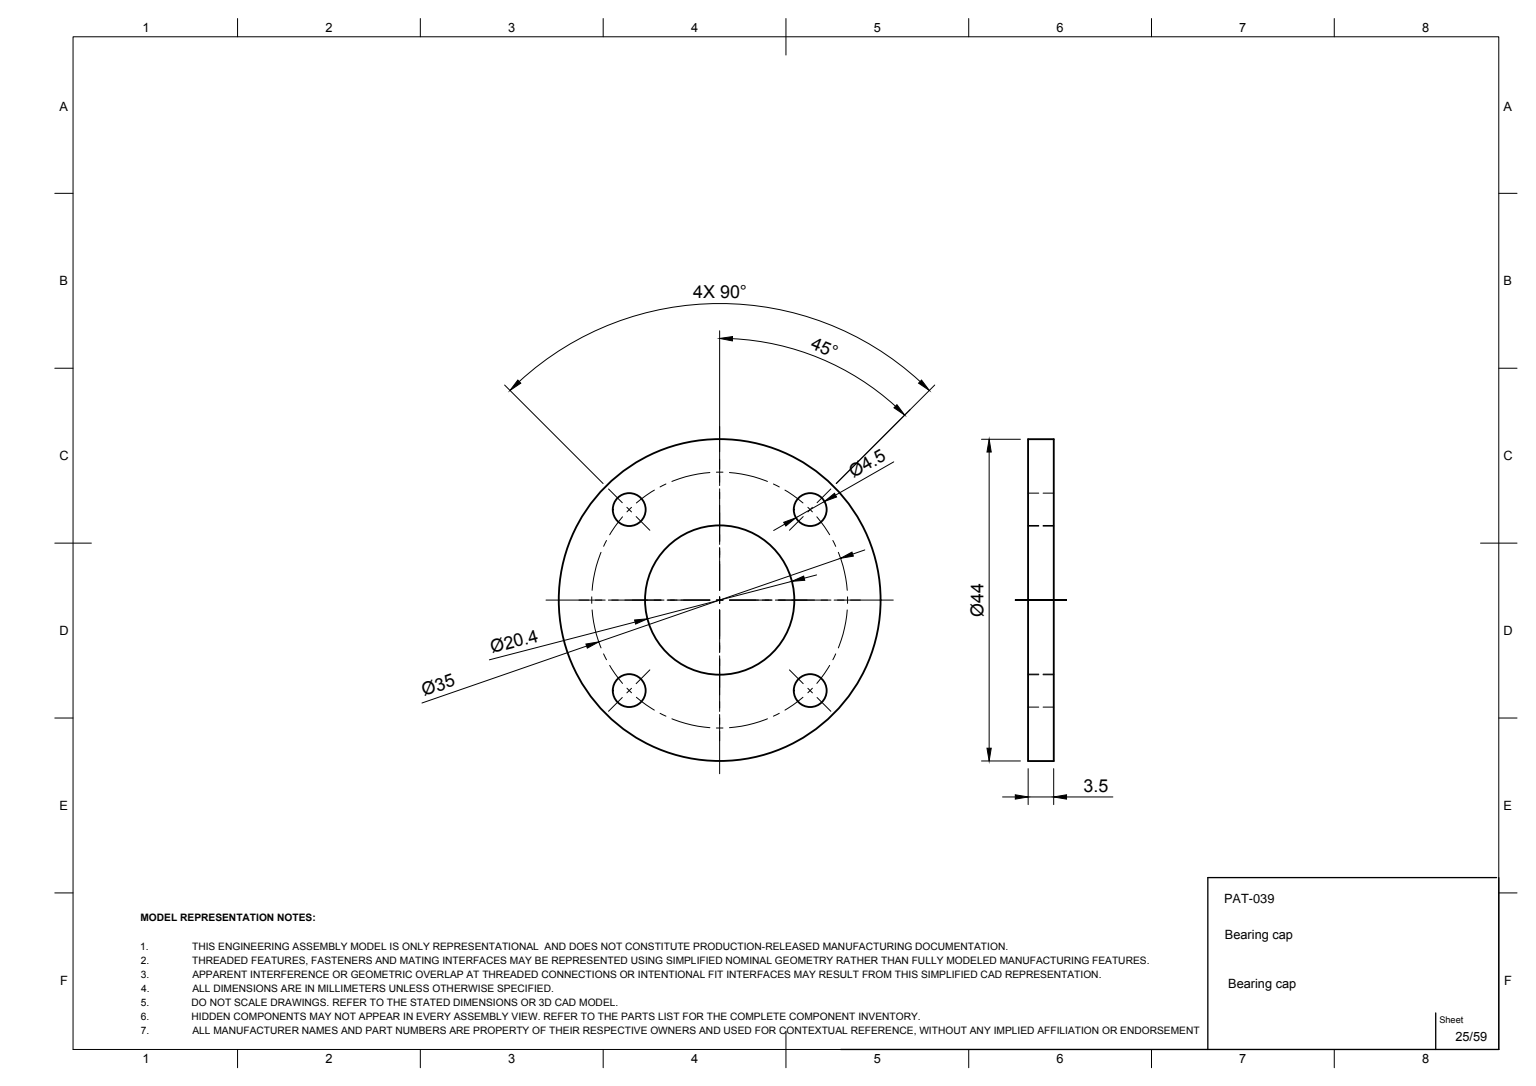
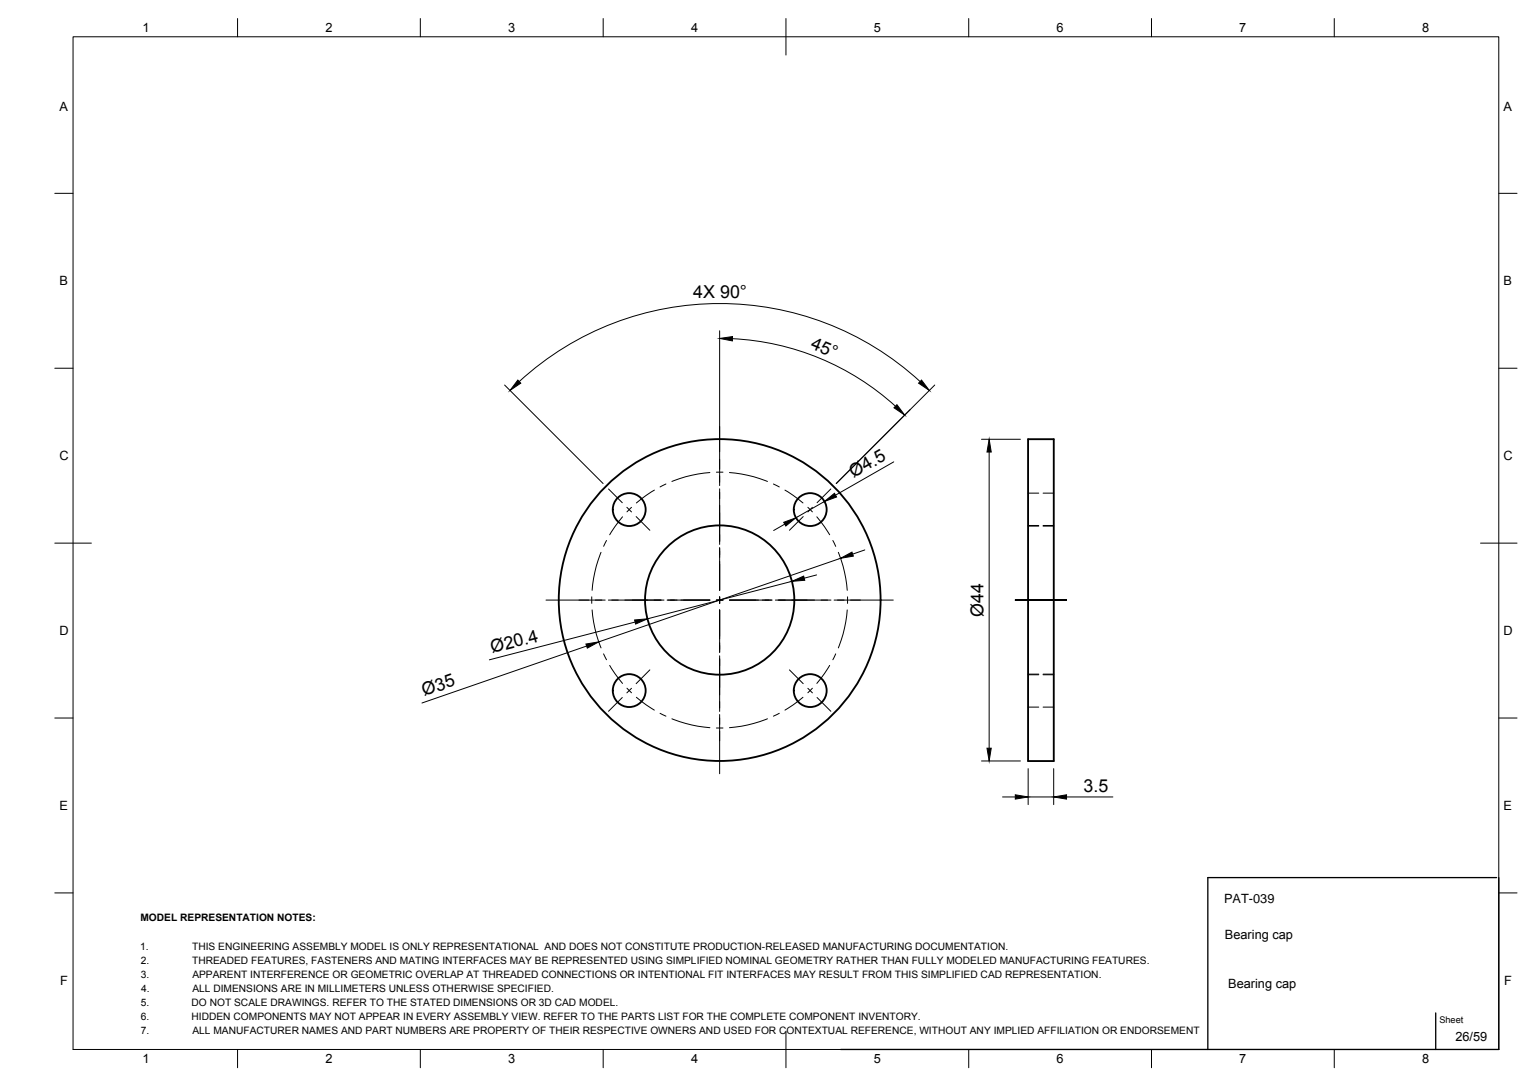
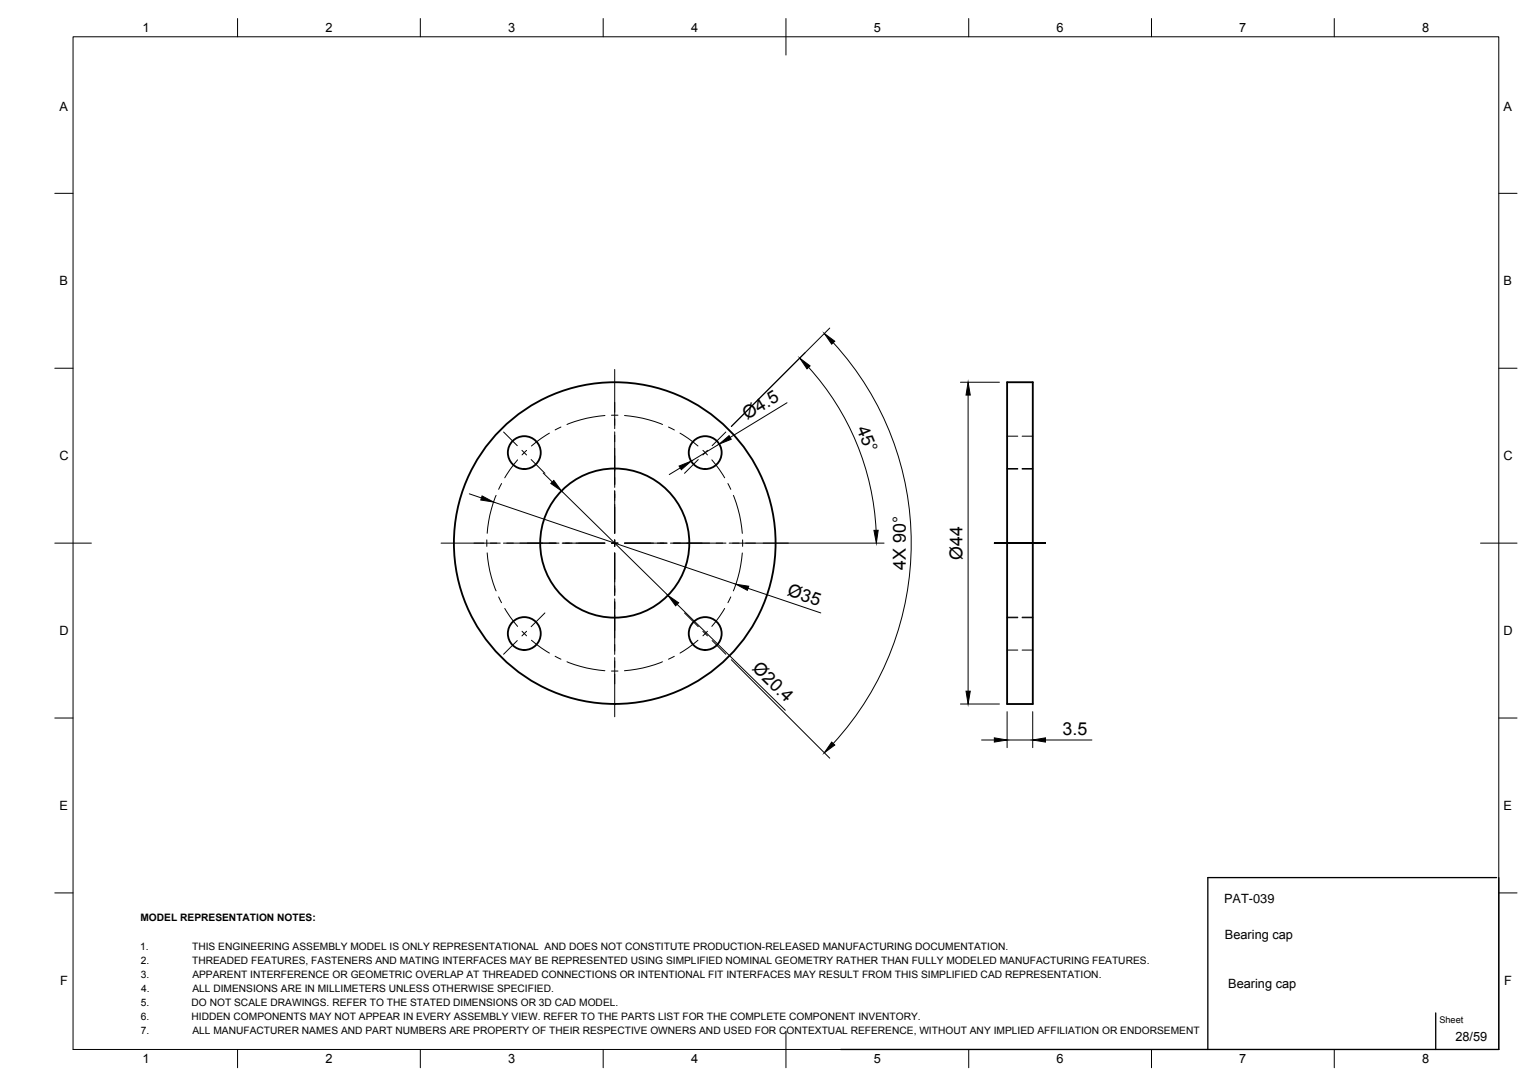
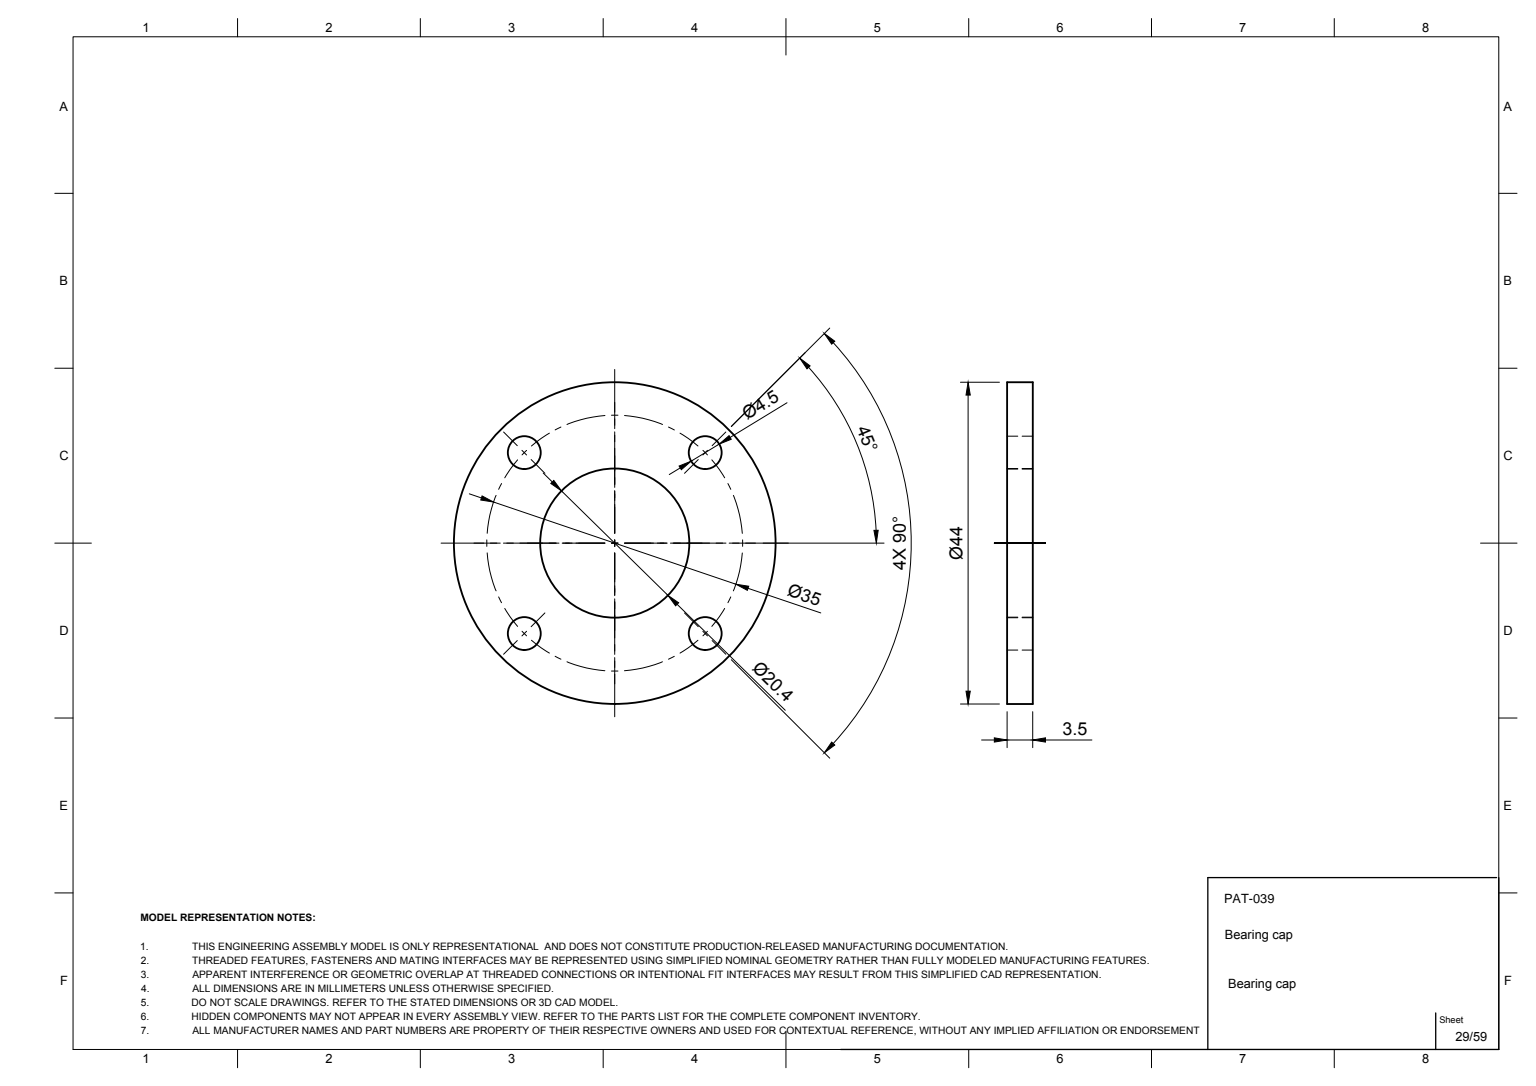
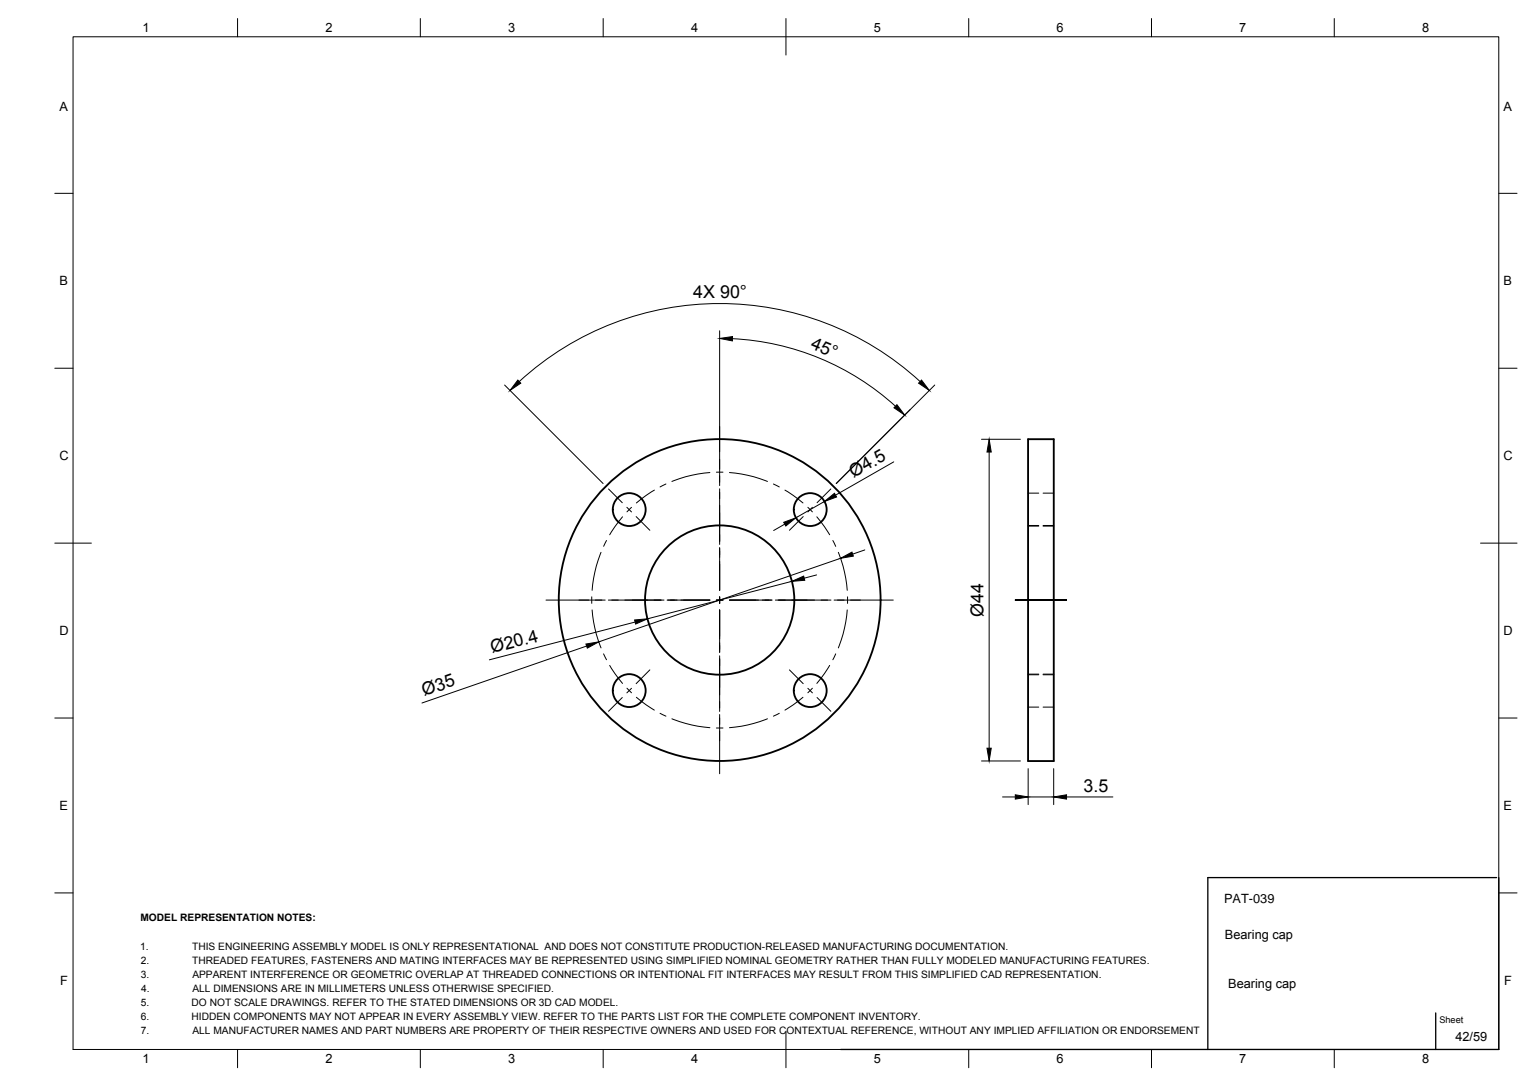
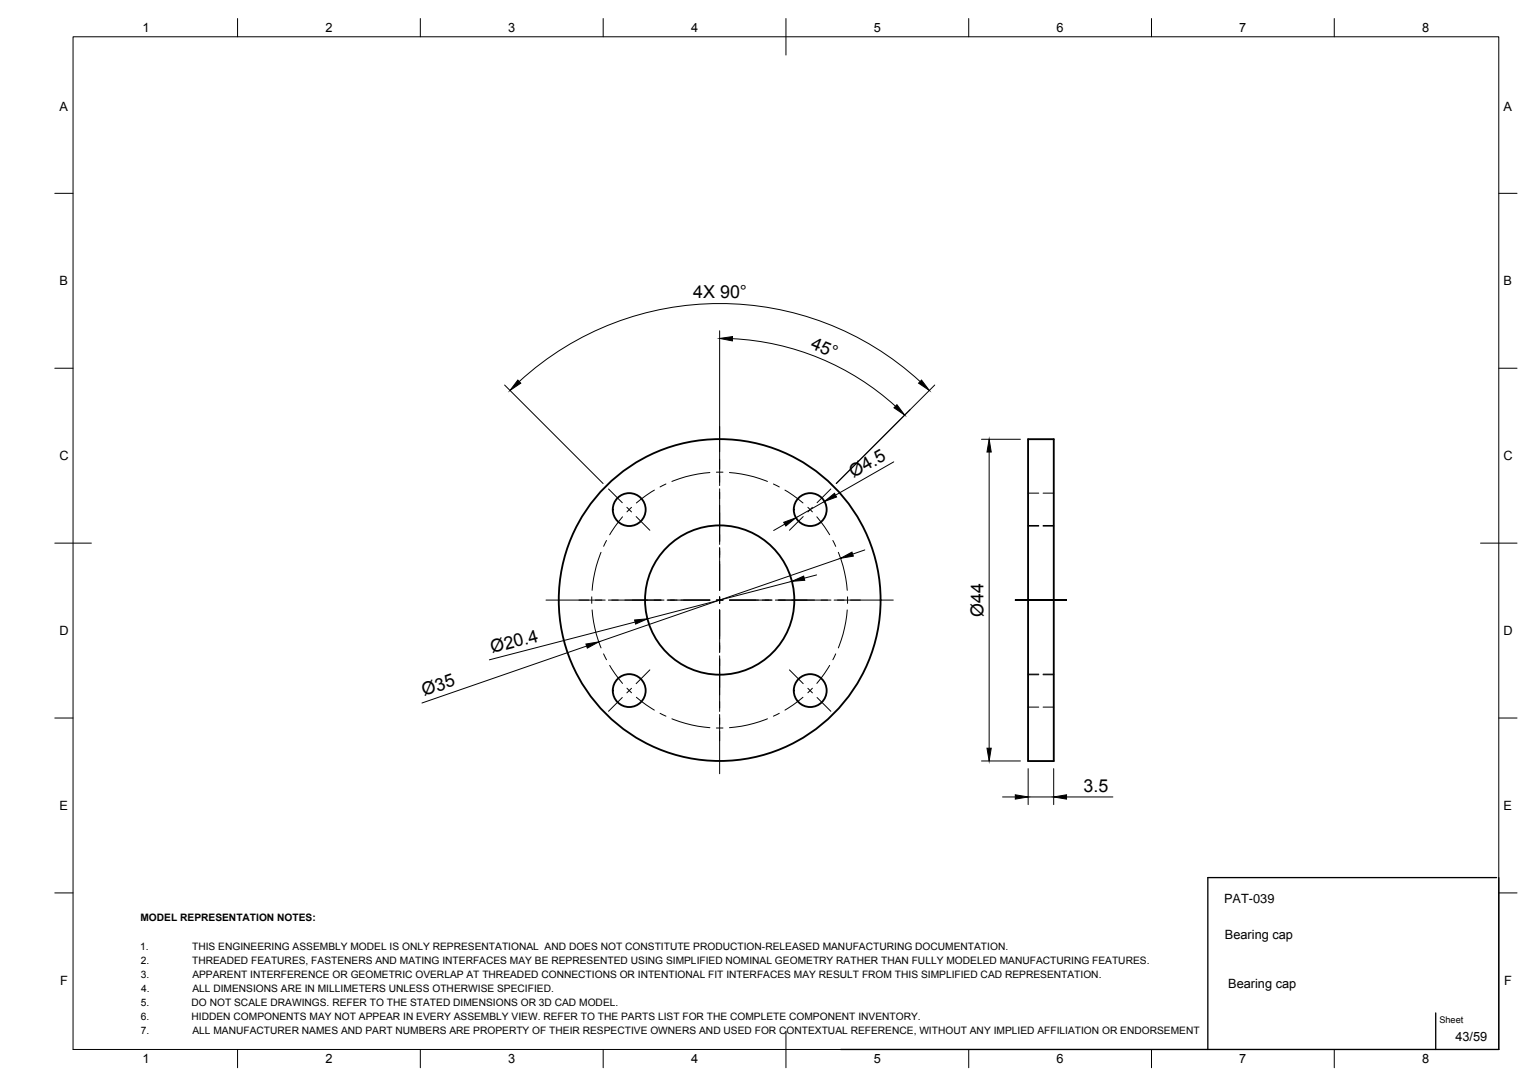
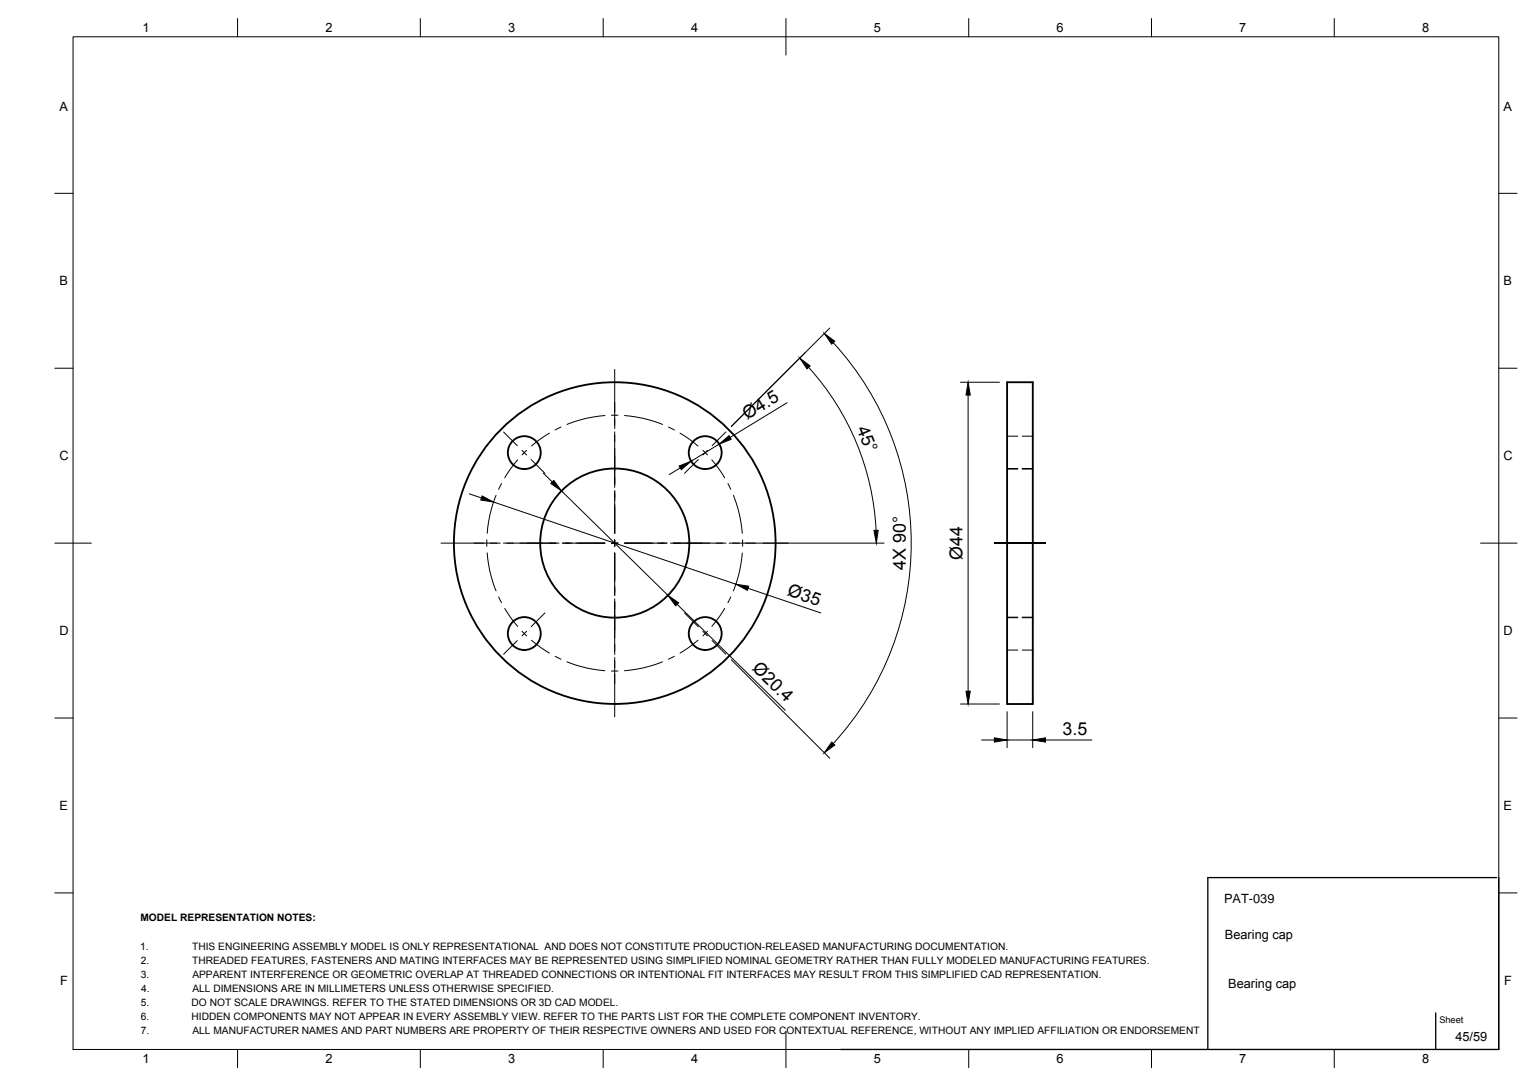
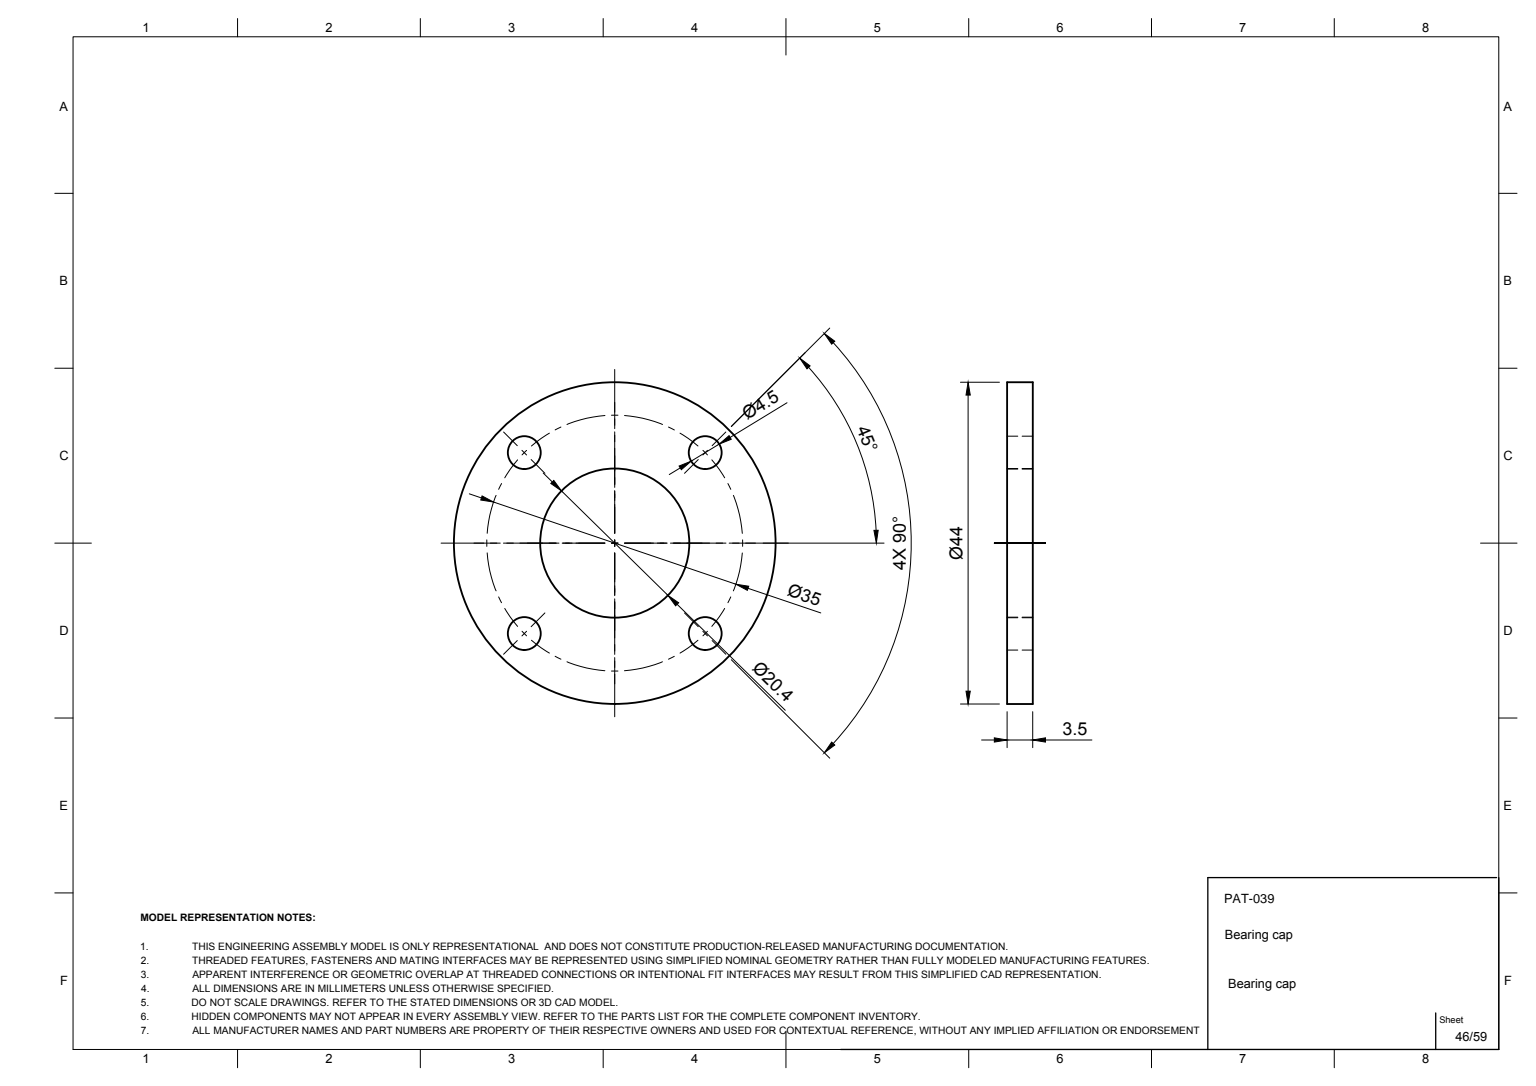
ISO-10303-21;
HEADER;
/* Generated by software containing ST-Developer
 * from STEP Tools, Inc. (www.steptools.com) 
 */

FILE_DESCRIPTION(
/* description */ ('Four-bar parallelogram arm'),
/* implementation_level */ '2;1');

FILE_NAME(
/* name */ 'Bearing cap.step',
/* time_stamp */ '2026-10-28T03:24:55-07:00',
/* author */ (''),
/* organization */ (''),
/* preprocessor_version */ 'ST-DEVELOPER v20.2',
/* originating_system */ 'Autodesk Translation Framework v15.17.0.0',
/* authorisation */ '');

FILE_SCHEMA (('AUTOMOTIVE_DESIGN { 1 0 10303 214 3 1 1 }'));
ENDSEC;

DATA;
#10=MECHANICAL_DESIGN_GEOMETRIC_PRESENTATION_REPRESENTATION('',(#641),#14512);
#541=SHAPE_REPRESENTATION_RELATIONSHIP('SRR','None',#14763,#591);
#591=ADVANCED_BREP_SHAPE_REPRESENTATION('',(#698),#14478);
#641=STYLED_ITEM('',(#15087),#698);
#698=MANIFOLD_SOLID_BREP('Body1',#7346);
#829=FACE_BOUND('',#1882,.T.);
#830=FACE_BOUND('',#1883,.T.);
#831=FACE_BOUND('',#1884,.T.);
#832=FACE_BOUND('',#1885,.T.);
#833=FACE_BOUND('',#1886,.T.);
#834=FACE_BOUND('',#1888,.T.);
#835=FACE_BOUND('',#1889,.T.);
#836=FACE_BOUND('',#1890,.T.);
#837=FACE_BOUND('',#1891,.T.);
#838=FACE_BOUND('',#1892,.T.);
#1095=PLANE('',#8278);
#1096=PLANE('',#8279);
#1361=FACE_OUTER_BOUND('',#1875,.T.);
#1362=FACE_OUTER_BOUND('',#1876,.T.);
#1363=FACE_OUTER_BOUND('',#1877,.T.);
#1364=FACE_OUTER_BOUND('',#1878,.T.);
#1365=FACE_OUTER_BOUND('',#1879,.T.);
#1366=FACE_OUTER_BOUND('',#1880,.T.);
#1367=FACE_OUTER_BOUND('',#1881,.T.);
#1368=FACE_OUTER_BOUND('',#1887,.T.);
#1875=EDGE_LOOP('',(#5646,#5647,#5648,#5649));
#1876=EDGE_LOOP('',(#5650,#5651,#5652,#5653));
#1877=EDGE_LOOP('',(#5654,#5655,#5656,#5657));
#1878=EDGE_LOOP('',(#5658,#5659,#5660,#5661));
#1879=EDGE_LOOP('',(#5662,#5663,#5664,#5665));
#1880=EDGE_LOOP('',(#5666,#5667,#5668,#5669));
#1881=EDGE_LOOP('',(#5670));
#1882=EDGE_LOOP('',(#5671));
#1883=EDGE_LOOP('',(#5672));
#1884=EDGE_LOOP('',(#5673));
#1885=EDGE_LOOP('',(#5674));
#1886=EDGE_LOOP('',(#5675));
#1887=EDGE_LOOP('',(#5676));
#1888=EDGE_LOOP('',(#5677));
#1889=EDGE_LOOP('',(#5678));
#1890=EDGE_LOOP('',(#5679));
#1891=EDGE_LOOP('',(#5680));
#1892=EDGE_LOOP('',(#5681));
#2495=LINE('',#12763,#2889);
#2496=LINE('',#12769,#2890);
#2497=LINE('',#12775,#2891);
#2498=LINE('',#12781,#2892);
#2499=LINE('',#12787,#2893);
#2500=LINE('',#12793,#2894);
#2889=VECTOR('',#9801,0.225);
#2890=VECTOR('',#9808,0.225);
#2891=VECTOR('',#9815,0.225);
#2892=VECTOR('',#9822,0.225);
#2893=VECTOR('',#9829,1.02);
#2894=VECTOR('',#9836,2.2);
#3240=CIRCLE('',#8261,0.225);
#3241=CIRCLE('',#8262,0.225);
#3242=CIRCLE('',#8264,0.225);
#3243=CIRCLE('',#8265,0.225);
#3244=CIRCLE('',#8267,0.225);
#3245=CIRCLE('',#8268,0.225);
#3246=CIRCLE('',#8270,0.225);
#3247=CIRCLE('',#8271,0.225);
#3248=CIRCLE('',#8273,1.02);
#3249=CIRCLE('',#8274,1.02);
#3250=CIRCLE('',#8276,2.2);
#3251=CIRCLE('',#8277,2.2);
#3762=VERTEX_POINT('',#12760);
#3763=VERTEX_POINT('',#12762);
#3764=VERTEX_POINT('',#12766);
#3765=VERTEX_POINT('',#12768);
#3766=VERTEX_POINT('',#12772);
#3767=VERTEX_POINT('',#12774);
#3768=VERTEX_POINT('',#12778);
#3769=VERTEX_POINT('',#12780);
#3770=VERTEX_POINT('',#12784);
#3771=VERTEX_POINT('',#12786);
#3772=VERTEX_POINT('',#12790);
#3773=VERTEX_POINT('',#12792);
#4454=EDGE_CURVE('',#3762,#3762,#3240,.T.);
#4455=EDGE_CURVE('',#3762,#3763,#2495,.T.);
#4456=EDGE_CURVE('',#3763,#3763,#3241,.T.);
#4457=EDGE_CURVE('',#3764,#3764,#3242,.T.);
#4458=EDGE_CURVE('',#3764,#3765,#2496,.T.);
#4459=EDGE_CURVE('',#3765,#3765,#3243,.T.);
#4460=EDGE_CURVE('',#3766,#3766,#3244,.T.);
#4461=EDGE_CURVE('',#3766,#3767,#2497,.T.);
#4462=EDGE_CURVE('',#3767,#3767,#3245,.T.);
#4463=EDGE_CURVE('',#3768,#3768,#3246,.T.);
#4464=EDGE_CURVE('',#3768,#3769,#2498,.T.);
#4465=EDGE_CURVE('',#3769,#3769,#3247,.T.);
#4466=EDGE_CURVE('',#3770,#3770,#3248,.T.);
#4467=EDGE_CURVE('',#3770,#3771,#2499,.T.);
#4468=EDGE_CURVE('',#3771,#3771,#3249,.T.);
#4469=EDGE_CURVE('',#3772,#3772,#3250,.T.);
#4470=EDGE_CURVE('',#3772,#3773,#2500,.T.);
#4471=EDGE_CURVE('',#3773,#3773,#3251,.T.);
#5646=ORIENTED_EDGE('',*,*,#4454,.F.);
#5647=ORIENTED_EDGE('',*,*,#4455,.T.);
#5648=ORIENTED_EDGE('',*,*,#4456,.F.);
#5649=ORIENTED_EDGE('',*,*,#4455,.F.);
#5650=ORIENTED_EDGE('',*,*,#4457,.F.);
#5651=ORIENTED_EDGE('',*,*,#4458,.T.);
#5652=ORIENTED_EDGE('',*,*,#4459,.F.);
#5653=ORIENTED_EDGE('',*,*,#4458,.F.);
#5654=ORIENTED_EDGE('',*,*,#4460,.F.);
#5655=ORIENTED_EDGE('',*,*,#4461,.T.);
#5656=ORIENTED_EDGE('',*,*,#4462,.F.);
#5657=ORIENTED_EDGE('',*,*,#4461,.F.);
#5658=ORIENTED_EDGE('',*,*,#4463,.F.);
#5659=ORIENTED_EDGE('',*,*,#4464,.T.);
#5660=ORIENTED_EDGE('',*,*,#4465,.F.);
#5661=ORIENTED_EDGE('',*,*,#4464,.F.);
#5662=ORIENTED_EDGE('',*,*,#4466,.F.);
#5663=ORIENTED_EDGE('',*,*,#4467,.T.);
#5664=ORIENTED_EDGE('',*,*,#4468,.T.);
#5665=ORIENTED_EDGE('',*,*,#4467,.F.);
#5666=ORIENTED_EDGE('',*,*,#4469,.F.);
#5667=ORIENTED_EDGE('',*,*,#4470,.T.);
#5668=ORIENTED_EDGE('',*,*,#4471,.T.);
#5669=ORIENTED_EDGE('',*,*,#4470,.F.);
#5670=ORIENTED_EDGE('',*,*,#4469,.T.);
#5671=ORIENTED_EDGE('',*,*,#4466,.T.);
#5672=ORIENTED_EDGE('',*,*,#4465,.T.);
#5673=ORIENTED_EDGE('',*,*,#4462,.T.);
#5674=ORIENTED_EDGE('',*,*,#4459,.T.);
#5675=ORIENTED_EDGE('',*,*,#4456,.T.);
#5676=ORIENTED_EDGE('',*,*,#4471,.F.);
#5677=ORIENTED_EDGE('',*,*,#4468,.F.);
#5678=ORIENTED_EDGE('',*,*,#4463,.T.);
#5679=ORIENTED_EDGE('',*,*,#4460,.T.);
#5680=ORIENTED_EDGE('',*,*,#4457,.T.);
#5681=ORIENTED_EDGE('',*,*,#4454,.T.);
#6781=CYLINDRICAL_SURFACE('',#8260,0.225);
#6782=CYLINDRICAL_SURFACE('',#8263,0.225);
#6783=CYLINDRICAL_SURFACE('',#8266,0.225);
#6784=CYLINDRICAL_SURFACE('',#8269,0.225);
#6785=CYLINDRICAL_SURFACE('',#8272,1.02);
#6786=CYLINDRICAL_SURFACE('',#8275,2.2);
#7066=ADVANCED_FACE('',(#1361),#6781,.F.);
#7067=ADVANCED_FACE('',(#1362),#6782,.F.);
#7068=ADVANCED_FACE('',(#1363),#6783,.F.);
#7069=ADVANCED_FACE('',(#1364),#6784,.F.);
#7070=ADVANCED_FACE('',(#1365),#6785,.F.);
#7071=ADVANCED_FACE('',(#1366),#6786,.T.);
#7072=ADVANCED_FACE('',(#1367,#829,#830,#831,#832,#833),#1095,.T.);
#7073=ADVANCED_FACE('',(#1368,#834,#835,#836,#837,#838),#1096,.F.);
#7346=CLOSED_SHELL('',(#7066,#7067,#7068,#7069,#7070,#7071,#7072,#7073));
#8259=AXIS2_PLACEMENT_3D('',#12758,#9795,#9796);
#8260=AXIS2_PLACEMENT_3D('',#12759,#9797,#9798);
#8261=AXIS2_PLACEMENT_3D('',#12761,#9799,#9800);
#8262=AXIS2_PLACEMENT_3D('',#12764,#9802,#9803);
#8263=AXIS2_PLACEMENT_3D('',#12765,#9804,#9805);
#8264=AXIS2_PLACEMENT_3D('',#12767,#9806,#9807);
#8265=AXIS2_PLACEMENT_3D('',#12770,#9809,#9810);
#8266=AXIS2_PLACEMENT_3D('',#12771,#9811,#9812);
#8267=AXIS2_PLACEMENT_3D('',#12773,#9813,#9814);
#8268=AXIS2_PLACEMENT_3D('',#12776,#9816,#9817);
#8269=AXIS2_PLACEMENT_3D('',#12777,#9818,#9819);
#8270=AXIS2_PLACEMENT_3D('',#12779,#9820,#9821);
#8271=AXIS2_PLACEMENT_3D('',#12782,#9823,#9824);
#8272=AXIS2_PLACEMENT_3D('',#12783,#9825,#9826);
#8273=AXIS2_PLACEMENT_3D('',#12785,#9827,#9828);
#8274=AXIS2_PLACEMENT_3D('',#12788,#9830,#9831);
#8275=AXIS2_PLACEMENT_3D('',#12789,#9832,#9833);
#8276=AXIS2_PLACEMENT_3D('',#12791,#9834,#9835);
#8277=AXIS2_PLACEMENT_3D('',#12794,#9837,#9838);
#8278=AXIS2_PLACEMENT_3D('',#12795,#9839,#9840);
#8279=AXIS2_PLACEMENT_3D('',#12796,#9841,#9842);
#9795=DIRECTION('axis',(0.,0.,1.));
#9796=DIRECTION('refdir',(1.,0.,0.));
#9797=DIRECTION('center_axis',(0.,1.,0.));
#9798=DIRECTION('ref_axis',(1.,0.,0.));
#9799=DIRECTION('center_axis',(0.,1.,0.));
#9800=DIRECTION('ref_axis',(1.,0.,0.));
#9801=DIRECTION('',(0.,1.,0.));
#9802=DIRECTION('center_axis',(0.,-1.,0.));
#9803=DIRECTION('ref_axis',(1.,0.,0.));
#9804=DIRECTION('center_axis',(0.,1.,0.));
#9805=DIRECTION('ref_axis',(1.,0.,0.));
#9806=DIRECTION('center_axis',(0.,1.,0.));
#9807=DIRECTION('ref_axis',(1.,0.,0.));
#9808=DIRECTION('',(0.,1.,0.));
#9809=DIRECTION('center_axis',(0.,-1.,0.));
#9810=DIRECTION('ref_axis',(1.,0.,0.));
#9811=DIRECTION('center_axis',(0.,1.,0.));
#9812=DIRECTION('ref_axis',(1.,0.,0.));
#9813=DIRECTION('center_axis',(0.,1.,0.));
#9814=DIRECTION('ref_axis',(1.,0.,0.));
#9815=DIRECTION('',(0.,1.,0.));
#9816=DIRECTION('center_axis',(0.,-1.,0.));
#9817=DIRECTION('ref_axis',(1.,0.,0.));
#9818=DIRECTION('center_axis',(0.,1.,0.));
#9819=DIRECTION('ref_axis',(1.,0.,0.));
#9820=DIRECTION('center_axis',(0.,1.,0.));
#9821=DIRECTION('ref_axis',(1.,0.,0.));
#9822=DIRECTION('',(0.,1.,0.));
#9823=DIRECTION('center_axis',(0.,-1.,0.));
#9824=DIRECTION('ref_axis',(1.,0.,0.));
#9825=DIRECTION('center_axis',(0.,1.,0.));
#9826=DIRECTION('ref_axis',(1.,0.,0.));
#9827=DIRECTION('center_axis',(0.,-1.,0.));
#9828=DIRECTION('ref_axis',(1.,0.,0.));
#9829=DIRECTION('',(0.,-1.,0.));
#9830=DIRECTION('center_axis',(0.,-1.,0.));
#9831=DIRECTION('ref_axis',(1.,0.,0.));
#9832=DIRECTION('center_axis',(0.,1.,0.));
#9833=DIRECTION('ref_axis',(1.,0.,0.));
#9834=DIRECTION('center_axis',(0.,1.,0.));
#9835=DIRECTION('ref_axis',(1.,0.,0.));
#9836=DIRECTION('',(0.,-1.,0.));
#9837=DIRECTION('center_axis',(0.,1.,0.));
#9838=DIRECTION('ref_axis',(1.,0.,0.));
#9839=DIRECTION('center_axis',(0.,1.,0.));
#9840=DIRECTION('ref_axis',(1.,0.,0.));
#9841=DIRECTION('center_axis',(0.,1.,0.));
#9842=DIRECTION('ref_axis',(1.,0.,0.));
#12758=CARTESIAN_POINT('',(0.,0.,0.));
#12759=CARTESIAN_POINT('Origin',(-1.23743686707646,-1.5,6.76256313292354));
#12760=CARTESIAN_POINT('',(-1.46243686707646,-1.4,6.76256313292354));
#12761=CARTESIAN_POINT('Origin',(-1.23743686707646,-1.4,6.76256313292354));
#12762=CARTESIAN_POINT('',(-1.46243686707646,-1.05,6.76256313292354));
#12763=CARTESIAN_POINT('',(-1.46243686707646,-1.5,6.76256313292354));
#12764=CARTESIAN_POINT('Origin',(-1.23743686707646,-1.05,6.76256313292354));
#12765=CARTESIAN_POINT('Origin',(-1.23743686707646,-1.5,9.23743686707646));
#12766=CARTESIAN_POINT('',(-1.46243686707646,-1.4,9.23743686707646));
#12767=CARTESIAN_POINT('Origin',(-1.23743686707646,-1.4,9.23743686707646));
#12768=CARTESIAN_POINT('',(-1.46243686707646,-1.05,9.23743686707646));
#12769=CARTESIAN_POINT('',(-1.46243686707646,-1.5,9.23743686707646));
#12770=CARTESIAN_POINT('Origin',(-1.23743686707646,-1.05,9.23743686707646));
#12771=CARTESIAN_POINT('Origin',(1.23743686707646,-1.5,9.23743686707646));
#12772=CARTESIAN_POINT('',(1.01243686707646,-1.4,9.23743686707646));
#12773=CARTESIAN_POINT('Origin',(1.23743686707646,-1.4,9.23743686707646));
#12774=CARTESIAN_POINT('',(1.01243686707646,-1.05,9.23743686707646));
#12775=CARTESIAN_POINT('',(1.01243686707646,-1.5,9.23743686707646));
#12776=CARTESIAN_POINT('Origin',(1.23743686707646,-1.05,9.23743686707646));
#12777=CARTESIAN_POINT('Origin',(1.23743686707646,-1.5,6.76256313292354));
#12778=CARTESIAN_POINT('',(1.01243686707646,-1.4,6.76256313292354));
#12779=CARTESIAN_POINT('Origin',(1.23743686707646,-1.4,6.76256313292354));
#12780=CARTESIAN_POINT('',(1.01243686707646,-1.05,6.76256313292354));
#12781=CARTESIAN_POINT('',(1.01243686707646,-1.5,6.76256313292354));
#12782=CARTESIAN_POINT('Origin',(1.23743686707646,-1.05,6.76256313292354));
#12783=CARTESIAN_POINT('Origin',(0.,-1.4,8.));
#12784=CARTESIAN_POINT('',(-1.02,-1.05,8.));
#12785=CARTESIAN_POINT('Origin',(0.,-1.05,8.));
#12786=CARTESIAN_POINT('',(-1.02,-1.4,8.));
#12787=CARTESIAN_POINT('',(-1.02,-1.4,8.));
#12788=CARTESIAN_POINT('Origin',(0.,-1.4,8.));
#12789=CARTESIAN_POINT('Origin',(0.,-1.4,8.));
#12790=CARTESIAN_POINT('',(-2.2,-1.05,8.));
#12791=CARTESIAN_POINT('Origin',(0.,-1.05,8.));
#12792=CARTESIAN_POINT('',(-2.2,-1.4,8.));
#12793=CARTESIAN_POINT('',(-2.2,-1.4,8.));
#12794=CARTESIAN_POINT('Origin',(0.,-1.4,8.));
#12795=CARTESIAN_POINT('Origin',(0.,-1.05,8.));
#12796=CARTESIAN_POINT('Origin',(0.,-1.4,8.));
#14421=UNCERTAINTY_MEASURE_WITH_UNIT(LENGTH_MEASURE(0.001),#14513,
'DISTANCE_ACCURACY_VALUE',
'Maximum model space distance between geometric entities at asserted c
onnectivities');
#14455=UNCERTAINTY_MEASURE_WITH_UNIT(LENGTH_MEASURE(0.001),#14513,
'DISTANCE_ACCURACY_VALUE',
'Maximum model space distance between geometric entities at asserted c
onnectivities');
#14478=(
GEOMETRIC_REPRESENTATION_CONTEXT(3)
GLOBAL_UNCERTAINTY_ASSIGNED_CONTEXT((#14421))
GLOBAL_UNIT_ASSIGNED_CONTEXT((#14513,#14515,#14516))
REPRESENTATION_CONTEXT('','3D')
);
#14512=(
GEOMETRIC_REPRESENTATION_CONTEXT(3)
GLOBAL_UNCERTAINTY_ASSIGNED_CONTEXT((#14455))
GLOBAL_UNIT_ASSIGNED_CONTEXT((#14513,#14515,#14516))
REPRESENTATION_CONTEXT('','3D')
);
#14513=(
LENGTH_UNIT()
NAMED_UNIT(*)
SI_UNIT(.CENTI.,.METRE.)
);
#14515=(
NAMED_UNIT(*)
PLANE_ANGLE_UNIT()
SI_UNIT($,.RADIAN.)
);
#14516=(
NAMED_UNIT(*)
SI_UNIT($,.STERADIAN.)
SOLID_ANGLE_UNIT()
);
#14539=SHAPE_DEFINITION_REPRESENTATION(#14595,#14763);
#14595=PRODUCT_DEFINITION_SHAPE('',$,#14820);
#14763=SHAPE_REPRESENTATION('',(#8259),#14478);
#14797=PRODUCT_DEFINITION_CONTEXT('part definition',#14967,'design');
#14820=PRODUCT_DEFINITION('Bearing cap','Bearing cap',#14876,#14797);
#14876=PRODUCT_DEFINITION_FORMATION('',$,#14991);
#14967=APPLICATION_CONTEXT(
'Core Data for Automotive Mechanical Design Process');
#14968=PRODUCT_CONTEXT('part definition',#14967,'mechanical');
#14991=PRODUCT('Bearing cap','Bearing cap','Bearing cap',(#14968));
#15081=COLOUR_RGB('Grey',0.48,0.52,0.57);
#15082=FILL_AREA_STYLE_COLOUR('',#15081);
#15083=FILL_AREA_STYLE('',(#15082));
#15084=SURFACE_STYLE_FILL_AREA(#15083);
#15085=SURFACE_SIDE_STYLE('',(#15084));
#15086=SURFACE_STYLE_USAGE(.BOTH.,#15085);
#15087=PRESENTATION_STYLE_ASSIGNMENT((#15086));
ENDSEC;
END-ISO-10303-21;
